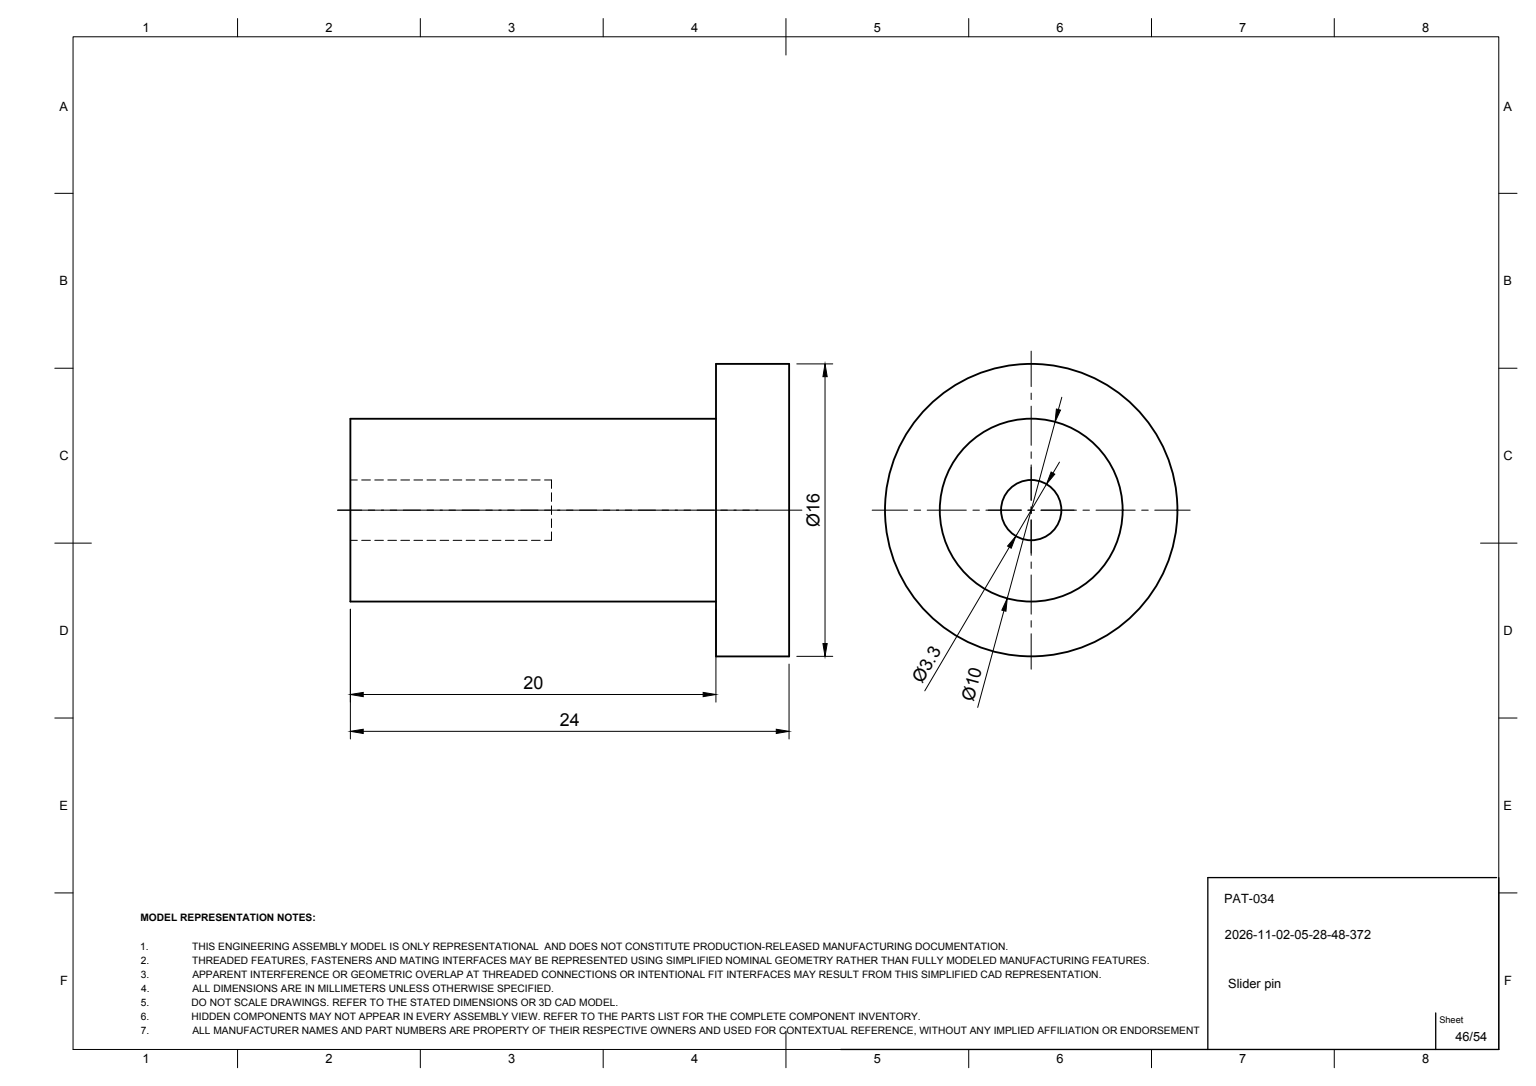
ISO-10303-21;
HEADER;
/* Generated by software containing ST-Developer
 * from STEP Tools, Inc. (www.steptools.com) 
 */

FILE_DESCRIPTION(
/* description */ ('Fatigue rig crank-slider'),
/* implementation_level */ '2;1');

FILE_NAME(
/* name */ 'Slider pin.step',
/* time_stamp */ '2026-10-28T03:24:50-07:00',
/* author */ (''),
/* organization */ (''),
/* preprocessor_version */ 'ST-DEVELOPER v20.2',
/* originating_system */ 'Autodesk Translation Framework v15.17.0.0',
/* authorisation */ '');

FILE_SCHEMA (('AUTOMOTIVE_DESIGN { 1 0 10303 214 3 1 1 }'));
ENDSEC;

DATA;
#10=MECHANICAL_DESIGN_GEOMETRIC_PRESENTATION_REPRESENTATION('',(#635),#16911);
#526=SHAPE_REPRESENTATION_RELATIONSHIP('SRR','None',#17170,#576);
#576=ADVANCED_BREP_SHAPE_REPRESENTATION('',(#692),#16899);
#635=STYLED_ITEM('',(#17487),#692);
#692=MANIFOLD_SOLID_BREP('Body1',#8928);
#880=FACE_BOUND('',#2331,.T.);
#881=FACE_BOUND('',#2336,.T.);
#1134=PLANE('',#10304);
#1135=PLANE('',#10305);
#1136=PLANE('',#10310);
#1137=PLANE('',#10313);
#1625=FACE_OUTER_BOUND('',#2328,.T.);
#1626=FACE_OUTER_BOUND('',#2329,.T.);
#1627=FACE_OUTER_BOUND('',#2330,.T.);
#1628=FACE_OUTER_BOUND('',#2332,.T.);
#1629=FACE_OUTER_BOUND('',#2333,.T.);
#1630=FACE_OUTER_BOUND('',#2334,.T.);
#1631=FACE_OUTER_BOUND('',#2335,.T.);
#2328=EDGE_LOOP('',(#7702,#7703,#7704,#7705));
#2329=EDGE_LOOP('',(#7706));
#2330=EDGE_LOOP('',(#7707));
#2331=EDGE_LOOP('',(#7708));
#2332=EDGE_LOOP('',(#7709,#7710,#7711,#7712));
#2333=EDGE_LOOP('',(#7713));
#2334=EDGE_LOOP('',(#7714,#7715,#7716,#7717));
#2335=EDGE_LOOP('',(#7718));
#2336=EDGE_LOOP('',(#7719));
#2920=LINE('',#16186,#3566);
#2921=LINE('',#16196,#3567);
#2922=LINE('',#16202,#3568);
#3566=VECTOR('',#12646,0.164999999999999);
#3567=VECTOR('',#12659,0.800000000000001);
#3568=VECTOR('',#12668,0.5);
#4091=CIRCLE('',#10302,0.164999999999999);
#4092=CIRCLE('',#10303,0.164999999999999);
#4093=CIRCLE('',#10306,0.800000000000001);
#4094=CIRCLE('',#10307,0.5);
#4095=CIRCLE('',#10309,0.800000000000001);
#4096=CIRCLE('',#10312,0.5);
#4735=VERTEX_POINT('',#16183);
#4736=VERTEX_POINT('',#16185);
#4737=VERTEX_POINT('',#16190);
#4738=VERTEX_POINT('',#16192);
#4739=VERTEX_POINT('',#16195);
#4740=VERTEX_POINT('',#16200);
#5749=EDGE_CURVE('',#4735,#4735,#4091,.T.);
#5750=EDGE_CURVE('',#4735,#4736,#2920,.T.);
#5751=EDGE_CURVE('',#4736,#4736,#4092,.T.);
#5752=EDGE_CURVE('',#4737,#4737,#4093,.T.);
#5753=EDGE_CURVE('',#4738,#4738,#4094,.T.);
#5754=EDGE_CURVE('',#4737,#4739,#2921,.T.);
#5755=EDGE_CURVE('',#4739,#4739,#4095,.T.);
#5756=EDGE_CURVE('',#4740,#4740,#4096,.T.);
#5757=EDGE_CURVE('',#4740,#4738,#2922,.T.);
#7702=ORIENTED_EDGE('',*,*,#5749,.F.);
#7703=ORIENTED_EDGE('',*,*,#5750,.T.);
#7704=ORIENTED_EDGE('',*,*,#5751,.F.);
#7705=ORIENTED_EDGE('',*,*,#5750,.F.);
#7706=ORIENTED_EDGE('',*,*,#5749,.T.);
#7707=ORIENTED_EDGE('',*,*,#5752,.T.);
#7708=ORIENTED_EDGE('',*,*,#5753,.F.);
#7709=ORIENTED_EDGE('',*,*,#5752,.F.);
#7710=ORIENTED_EDGE('',*,*,#5754,.T.);
#7711=ORIENTED_EDGE('',*,*,#5755,.T.);
#7712=ORIENTED_EDGE('',*,*,#5754,.F.);
#7713=ORIENTED_EDGE('',*,*,#5755,.F.);
#7714=ORIENTED_EDGE('',*,*,#5756,.F.);
#7715=ORIENTED_EDGE('',*,*,#5757,.T.);
#7716=ORIENTED_EDGE('',*,*,#5753,.T.);
#7717=ORIENTED_EDGE('',*,*,#5757,.F.);
#7718=ORIENTED_EDGE('',*,*,#5756,.T.);
#7719=ORIENTED_EDGE('',*,*,#5751,.T.);
#8334=CYLINDRICAL_SURFACE('',#10301,0.164999999999999);
#8335=CYLINDRICAL_SURFACE('',#10308,0.800000000000001);
#8336=CYLINDRICAL_SURFACE('',#10311,0.5);
#8763=ADVANCED_FACE('',(#1625),#8334,.F.);
#8764=ADVANCED_FACE('',(#1626),#1134,.T.);
#8765=ADVANCED_FACE('',(#1627,#880),#1135,.T.);
#8766=ADVANCED_FACE('',(#1628),#8335,.T.);
#8767=ADVANCED_FACE('',(#1629),#1136,.F.);
#8768=ADVANCED_FACE('',(#1630),#8336,.T.);
#8769=ADVANCED_FACE('',(#1631,#881),#1137,.T.);
#8928=CLOSED_SHELL('',(#8763,#8764,#8765,#8766,#8767,#8768,#8769));
#10300=AXIS2_PLACEMENT_3D('',#16181,#12640,#12641);
#10301=AXIS2_PLACEMENT_3D('',#16182,#12642,#12643);
#10302=AXIS2_PLACEMENT_3D('',#16184,#12644,#12645);
#10303=AXIS2_PLACEMENT_3D('',#16187,#12647,#12648);
#10304=AXIS2_PLACEMENT_3D('',#16188,#12649,#12650);
#10305=AXIS2_PLACEMENT_3D('',#16189,#12651,#12652);
#10306=AXIS2_PLACEMENT_3D('',#16191,#12653,#12654);
#10307=AXIS2_PLACEMENT_3D('',#16193,#12655,#12656);
#10308=AXIS2_PLACEMENT_3D('',#16194,#12657,#12658);
#10309=AXIS2_PLACEMENT_3D('',#16197,#12660,#12661);
#10310=AXIS2_PLACEMENT_3D('',#16198,#12662,#12663);
#10311=AXIS2_PLACEMENT_3D('',#16199,#12664,#12665);
#10312=AXIS2_PLACEMENT_3D('',#16201,#12666,#12667);
#10313=AXIS2_PLACEMENT_3D('',#16203,#12669,#12670);
#12640=DIRECTION('axis',(0.,0.,1.));
#12641=DIRECTION('refdir',(1.,0.,0.));
#12642=DIRECTION('center_axis',(0.,1.,0.));
#12643=DIRECTION('ref_axis',(1.,0.,0.));
#12644=DIRECTION('center_axis',(0.,1.,0.));
#12645=DIRECTION('ref_axis',(1.,0.,0.));
#12646=DIRECTION('',(0.,1.,0.));
#12647=DIRECTION('center_axis',(0.,-1.,0.));
#12648=DIRECTION('ref_axis',(1.,0.,0.));
#12649=DIRECTION('center_axis',(0.,1.,0.));
#12650=DIRECTION('ref_axis',(1.,0.,0.));
#12651=DIRECTION('center_axis',(0.,1.,0.));
#12652=DIRECTION('ref_axis',(1.,0.,0.));
#12653=DIRECTION('center_axis',(0.,1.,0.));
#12654=DIRECTION('ref_axis',(1.,0.,0.));
#12655=DIRECTION('center_axis',(0.,1.,0.));
#12656=DIRECTION('ref_axis',(1.,0.,0.));
#12657=DIRECTION('center_axis',(0.,1.,0.));
#12658=DIRECTION('ref_axis',(1.,0.,0.));
#12659=DIRECTION('',(0.,-1.,0.));
#12660=DIRECTION('center_axis',(0.,1.,0.));
#12661=DIRECTION('ref_axis',(1.,0.,0.));
#12662=DIRECTION('center_axis',(0.,1.,0.));
#12663=DIRECTION('ref_axis',(1.,0.,0.));
#12664=DIRECTION('center_axis',(0.,1.,0.));
#12665=DIRECTION('ref_axis',(1.,0.,0.));
#12666=DIRECTION('center_axis',(0.,1.,0.));
#12667=DIRECTION('ref_axis',(1.,0.,0.));
#12668=DIRECTION('',(0.,-1.,0.));
#12669=DIRECTION('center_axis',(0.,1.,0.));
#12670=DIRECTION('ref_axis',(1.,0.,0.));
#16181=CARTESIAN_POINT('',(0.,0.,0.));
#16182=CARTESIAN_POINT('Origin',(11.,3.7,12.));
#16183=CARTESIAN_POINT('',(10.835,3.7,12.));
#16184=CARTESIAN_POINT('Origin',(11.,3.7,12.));
#16185=CARTESIAN_POINT('',(10.835,4.8,12.));
#16186=CARTESIAN_POINT('',(10.835,3.7,12.));
#16187=CARTESIAN_POINT('Origin',(11.,4.8,12.));
#16188=CARTESIAN_POINT('Origin',(11.,3.7,12.));
#16189=CARTESIAN_POINT('Origin',(11.,2.8,12.));
#16190=CARTESIAN_POINT('',(10.2,2.8,12.));
#16191=CARTESIAN_POINT('Origin',(11.,2.8,12.));
#16192=CARTESIAN_POINT('',(10.5,2.8,12.));
#16193=CARTESIAN_POINT('Origin',(11.,2.8,12.));
#16194=CARTESIAN_POINT('Origin',(11.,2.4,12.));
#16195=CARTESIAN_POINT('',(10.2,2.4,12.));
#16196=CARTESIAN_POINT('',(10.2,2.4,12.));
#16197=CARTESIAN_POINT('Origin',(11.,2.4,12.));
#16198=CARTESIAN_POINT('Origin',(11.,2.4,12.));
#16199=CARTESIAN_POINT('Origin',(11.,2.8,12.));
#16200=CARTESIAN_POINT('',(10.5,4.8,12.));
#16201=CARTESIAN_POINT('Origin',(11.,4.8,12.));
#16202=CARTESIAN_POINT('',(10.5,2.8,12.));
#16203=CARTESIAN_POINT('Origin',(11.,4.8,12.));
#16840=UNCERTAINTY_MEASURE_WITH_UNIT(LENGTH_MEASURE(0.001),#16912,
'DISTANCE_ACCURACY_VALUE',
'Maximum model space distance between geometric entities at asserted c
onnectivities');
#16852=UNCERTAINTY_MEASURE_WITH_UNIT(LENGTH_MEASURE(0.001),#16912,
'DISTANCE_ACCURACY_VALUE',
'Maximum model space distance between geometric entities at asserted c
onnectivities');
#16899=(
GEOMETRIC_REPRESENTATION_CONTEXT(3)
GLOBAL_UNCERTAINTY_ASSIGNED_CONTEXT((#16840))
GLOBAL_UNIT_ASSIGNED_CONTEXT((#16912,#16914,#16915))
REPRESENTATION_CONTEXT('','3D')
);
#16911=(
GEOMETRIC_REPRESENTATION_CONTEXT(3)
GLOBAL_UNCERTAINTY_ASSIGNED_CONTEXT((#16852))
GLOBAL_UNIT_ASSIGNED_CONTEXT((#16912,#16914,#16915))
REPRESENTATION_CONTEXT('','3D')
);
#16912=(
LENGTH_UNIT()
NAMED_UNIT(*)
SI_UNIT(.CENTI.,.METRE.)
);
#16914=(
NAMED_UNIT(*)
PLANE_ANGLE_UNIT()
SI_UNIT($,.RADIAN.)
);
#16915=(
NAMED_UNIT(*)
SI_UNIT($,.STERADIAN.)
SOLID_ANGLE_UNIT()
);
#16962=SHAPE_DEFINITION_REPRESENTATION(#17034,#17170);
#17034=PRODUCT_DEFINITION_SHAPE('',$,#17229);
#17170=SHAPE_REPRESENTATION('',(#10300),#16899);
#17182=PRODUCT_DEFINITION_CONTEXT('part definition',#17358,'design');
#17229=PRODUCT_DEFINITION('Slider pin','Slider pin',#17287,#17182);
#17287=PRODUCT_DEFINITION_FORMATION('',$,#17406);
#17358=APPLICATION_CONTEXT(
'Core Data for Automotive Mechanical Design Process');
#17359=PRODUCT_CONTEXT('part definition',#17358,'mechanical');
#17406=PRODUCT('Slider pin','Slider pin','Slider pin',(#17359));
#17481=COLOUR_RGB('Grey',0.48,0.52,0.57);
#17482=FILL_AREA_STYLE_COLOUR('',#17481);
#17483=FILL_AREA_STYLE('',(#17482));
#17484=SURFACE_STYLE_FILL_AREA(#17483);
#17485=SURFACE_SIDE_STYLE('',(#17484));
#17486=SURFACE_STYLE_USAGE(.BOTH.,#17485);
#17487=PRESENTATION_STYLE_ASSIGNMENT((#17486));
ENDSEC;
END-ISO-10303-21;
